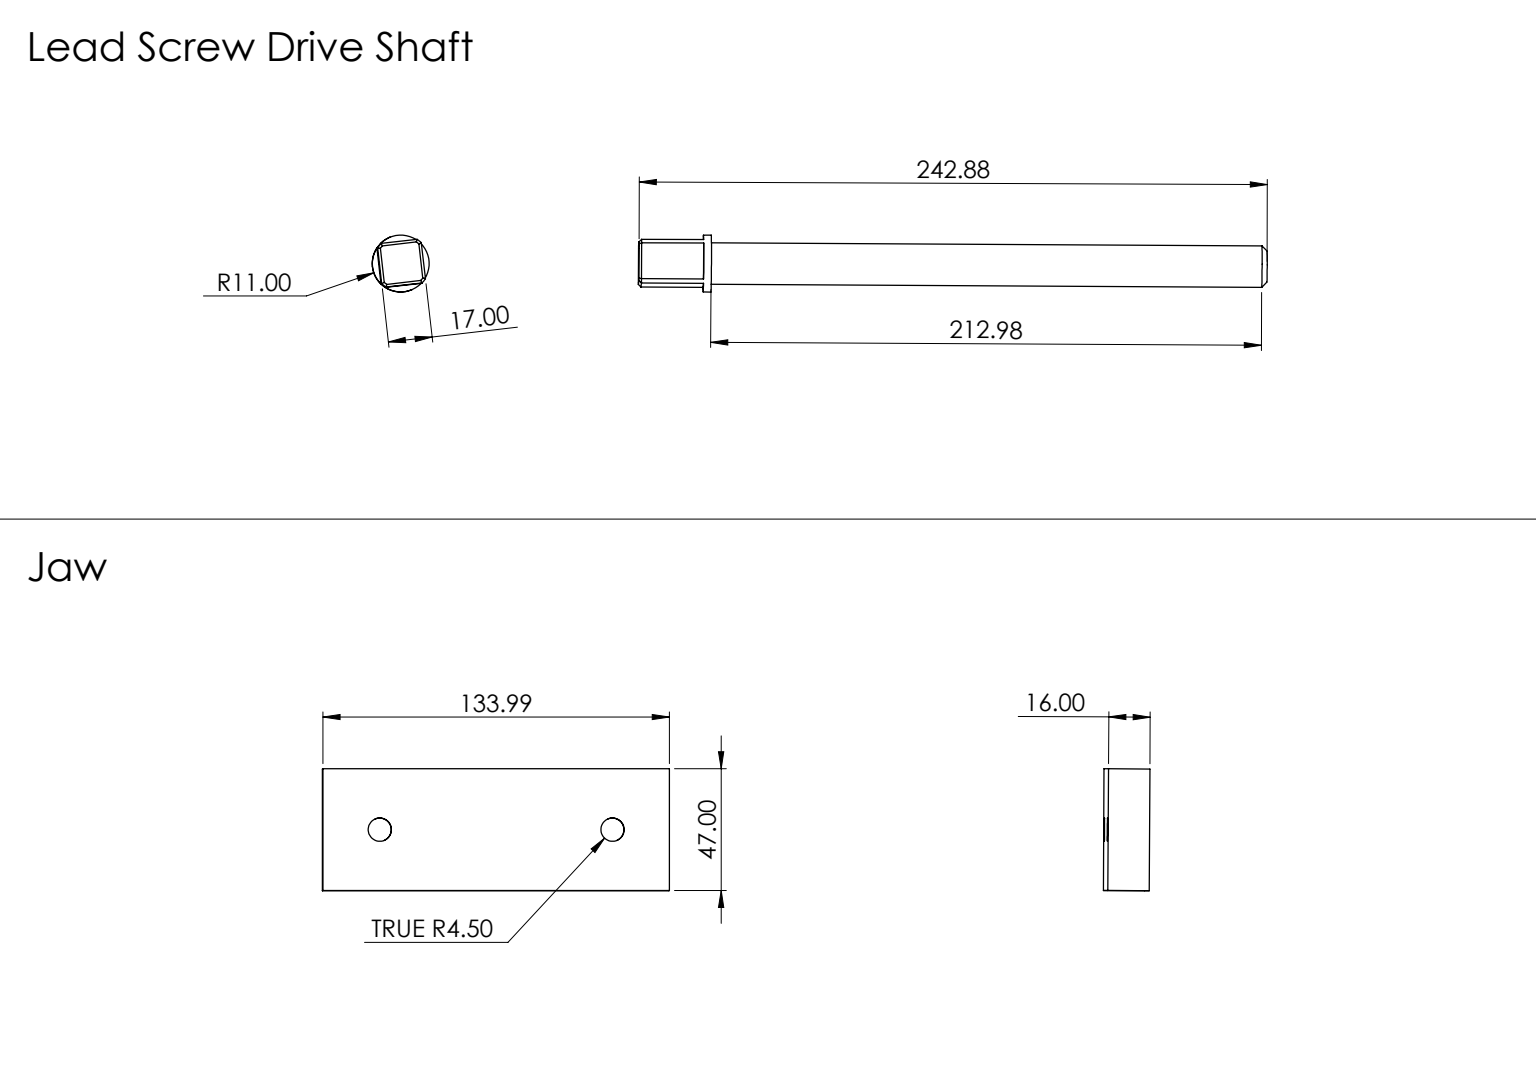
ISO-10303-21;
HEADER;
FILE_DESCRIPTION (('STEP AP214'),
    '1' );
FILE_NAME ('Lead Screw Drive Shaft.step',
    '2026-10-09T10:51:02',
    ( '' ),
    ( '' ),
    'SwSTEP 2.0',
    'SolidWorks 2026',
    '' );
FILE_SCHEMA (( 'AUTOMOTIVE_DESIGN' ));
ENDSEC;

DATA;
#4=CARTESIAN_POINT ( 'NONE',  ( 8.705884045762138257, 173.3519990577861734, 81.47578913282544022 ) ) ;
#29=EDGE_CURVE ( 'NONE', #2768, #16051, #13115, .T. ) ;
#43=AXIS2_PLACEMENT_3D ( 'NONE', #10674, #12520, #10452 ) ;
#64=DIRECTION ( 'NONE',  ( 0.9934404589540163366, 0.1135548637187051291, -0.01346653032743023830 ) ) ;
#93=EDGE_CURVE ( 'NONE', #564, #16051, #11405, .T. ) ;
#104=CIRCLE ( 'NONE', #1575, 11.00000000000000178 ) ;
#111=CARTESIAN_POINT ( 'NONE',  ( 11.83347885643962982, 174.6861507205185546, 323.4518999165990181 ) ) ;
#116=FACE_OUTER_BOUND ( 'NONE', #21594, .T. ) ;
#154=PLANE ( 'NONE',  #20182 ) ;
#206=ORIENTED_EDGE ( 'NONE', *, *, #693, .T. ) ;
#224=EDGE_LOOP ( 'NONE', ( #13231, #22623, #16630, #19910 ) ) ;
#250=DIRECTION ( 'NONE',  ( 0.01292394549866731669, 0.005513023399720593139, 0.9999012842304692006 ) ) ;
#260=DIRECTION ( 'NONE',  ( -0.9934404589540163366, -0.1135548637187053511, 0.01346653032743023309 ) ) ;
#279=FACE_BOUND ( 'NONE', #1045, .T. ) ;
#293=ORIENTED_EDGE ( 'NONE', *, *, #12181, .F. ) ;
#343=CARTESIAN_POINT ( 'NONE',  ( 11.77442667496907625, 158.9997348699313591, 299.5367818821357560 ) ) ;
#349=EDGE_CURVE ( 'NONE', #12132, #16568, #18988, .T. ) ;
#417=DIRECTION ( 'NONE',  ( 0.01292394549866731669, 0.005513023399720593139, 0.9999012842304692006 ) ) ;
#564=VERTEX_POINT ( 'NONE', #20430 ) ;
#595=ORIENTED_EDGE ( 'NONE', *, *, #9993, .F. ) ;
#640=CARTESIAN_POINT ( 'NONE',  ( 11.98277897518291013, 166.6990352492036891, 81.47011610648978319 ) ) ;
#646=CARTESIAN_POINT ( 'NONE',  ( 11.77702168924416171, 159.7711821663725971, 324.2021903088674435 ) ) ;
#675=ORIENTED_EDGE ( 'NONE', *, *, #17369, .T. ) ;
#693=EDGE_CURVE ( 'NONE', #2734, #11822, #9952, .T. ) ;
#712=EDGE_LOOP ( 'NONE', ( #4652, #19720, #8639 ) ) ;
#738=DIRECTION ( 'NONE',  ( 0.9934404589540163366, 0.1135548637187053511, -0.01346653032743023309 ) ) ;
#747=LINE ( 'NONE', #4054, #17299 ) ;
#771=PLANE ( 'NONE',  #14491 ) ;
#797=CIRCLE ( 'NONE', #1538, 11.00000000000000178 ) ;
#865=ORIENTED_EDGE ( 'NONE', *, *, #11226, .F. ) ;
#914=VECTOR ( 'NONE', #14909, 1000.000000000000114 ) ;
#942=FACE_OUTER_BOUND ( 'NONE', #11915, .T. ) ;
#1022=ORIENTED_EDGE ( 'NONE', *, *, #12685, .F. ) ;
#1045=EDGE_LOOP ( 'NONE', ( #20981, #3782 ) ) ;
#1078=ORIENTED_EDGE ( 'NONE', *, *, #12885, .T. ) ;
#1151=LINE ( 'NONE', #18927, #20877 ) ;
#1187=ORIENTED_EDGE ( 'NONE', *, *, #19016, .F. ) ;
#1189=CARTESIAN_POINT ( 'NONE',  ( -1.614838104868287605, 158.2404303229639595, 324.3837229658399792 ) ) ;
#1239=EDGE_CURVE ( 'NONE', #13001, #13489, #17742, .T. ) ;
#1325=VERTEX_POINT ( 'NONE', #16703 ) ;
#1384=PRODUCT_CONTEXT ( 'NONE', #22565, 'mechanical' ) ;
#1395=DIRECTION ( 'NONE',  ( 1.000000000000000000, 0.000000000000000000, 0.000000000000000000 ) ) ;
#1429=AXIS2_PLACEMENT_3D ( 'NONE', #11749, #10141, #6471 ) ;
#1438=DIRECTION ( 'NONE',  ( 0.01292394549866731843, 0.005513023399720594006, 0.9999012842304693116 ) ) ;
#1526=STYLED_ITEM ( 'NONE', ( #11230 ), #9502 ) ;
#1538=AXIS2_PLACEMENT_3D ( 'NONE', #8085, #15121, #22073 ) ;
#1544=CARTESIAN_POINT ( 'NONE',  ( 12.39776786404130782, 161.0697644098447370, 324.5197799491688215 ) ) ;
#1565=ADVANCED_FACE ( 'NONE', ( #19625 ), #12400, .T. ) ;
#1575=AXIS2_PLACEMENT_3D ( 'NONE', #11584, #21774, #9508 ) ;
#1609=CIRCLE ( 'NONE', #16669, 8.000000000000003553 ) ;
#1662=AXIS2_PLACEMENT_3D ( 'NONE', #19654, #14289, #2098 ) ;
#1701=CARTESIAN_POINT ( 'NONE',  ( 3.872354045398203937, 166.6517708494369856, 299.5967279023338392 ) ) ;
#1761=EDGE_CURVE ( 'NONE', #4814, #10791, #21560, .T. ) ;
#1791=ADVANCED_FACE ( 'NONE', ( #4229 ), #14606, .F. ) ;
#1795=CARTESIAN_POINT ( 'NONE',  ( -8.182603756456146016, 171.4215663745681866, 81.70472014839175756 ) ) ;
#1821=CARTESIAN_POINT ( 'NONE',  ( 3.872354045398203937, 166.6517708494369856, 299.5967279023338392 ) ) ;
#1838=CARTESIAN_POINT ( 'NONE',  ( 4.182528737366220106, 166.7840834110302808, 323.5943587238651276 ) ) ;
#1841=EDGE_CURVE ( 'NONE', #5715, #14396, #16176, .T. ) ;
#1848=CIRCLE ( 'NONE', #19071, 11.00000000000000178 ) ;
#1892=PRODUCT_DEFINITION_SHAPE ( 'NONE', 'NONE',  #18443 ) ;
#1900=AXIS2_PLACEMENT_3D ( 'NONE', #17981, #5764, #738 ) ;
#1903=CARTESIAN_POINT ( 'NONE',  ( 13.28235005706528682, 159.1720975239875884, 299.5163413053770682 ) ) ;
#1959=CIRCLE ( 'NONE', #13704, 10.00000000000005684 ) ;
#1987=CARTESIAN_POINT ( 'NONE',  ( 13.59252474903330210, 159.3044100855808836, 323.5139721269083566 ) ) ;
#1989=VERTEX_POINT ( 'NONE', #11897 ) ;
#2012=DIRECTION ( 'NONE',  ( -0.9934404589540163366, -0.1135548637187053511, 0.01346653032743023309 ) ) ;
#2016=ORIENTED_EDGE ( 'NONE', *, *, #19731, .F. ) ;
#2019=DIRECTION ( 'NONE',  ( -0.01292394549866731669, -0.005513023399720593139, -0.9999012842304692006 ) ) ;
#2022=ORIENTED_EDGE ( 'NONE', *, *, #9067, .T. ) ;
#2058=CARTESIAN_POINT ( 'NONE',  ( -4.905708827035327069, 164.7686025659857023, 81.69904712205610053 ) ) ;
#2082=ORIENTED_EDGE ( 'NONE', *, *, #20790, .F. ) ;
#2098=DIRECTION ( 'NONE',  ( -0.9934404589540177799, -0.1135548637186921672, 0.01346653032743275538 ) ) ;
#2175=VECTOR ( 'NONE', #10101, 1000.000000000000000 ) ;
#2192=CARTESIAN_POINT ( 'NONE',  ( 1.054933926688728762, 165.4499317482979279, 81.61824794009152129 ) ) ;
#2204=ORIENTED_EDGE ( 'NONE', *, *, #13338, .F. ) ;
#2244=VECTOR ( 'NONE', #7831, 1000.000000000000114 ) ;
#2266=ORIENTED_EDGE ( 'NONE', *, *, #14796, .T. ) ;
#2267=EDGE_LOOP ( 'NONE', ( #2022, #21934 ) ) ;
#2268=ORIENTED_EDGE ( 'NONE', *, *, #1239, .T. ) ;
#2283=DIRECTION ( 'NONE',  ( -0.1136178953597573732, 0.9935164314186356593, -0.004009283626633518283 ) ) ;
#2328=DIRECTION ( 'NONE',  ( 0.9934404589540162256, 0.1135548637187056842, -0.01346653032743081423 ) ) ;
#2356=EDGE_CURVE ( 'NONE', #6945, #13489, #4994, .T. ) ;
#2357=EDGE_CURVE ( 'NONE', #10791, #4814, #19010, .T. ) ;
#2442=CARTESIAN_POINT ( 'NONE',  ( 3.872354045398203937, 166.6517708494369856, 299.5967279023338392 ) ) ;
#2455=PLANE ( 'NONE',  #12630 ) ;
#2478=LINE ( 'NONE', #9473, #17026 ) ;
#2602=CARTESIAN_POINT ( 'NONE',  ( 11.61857788991896179, 160.0893180226940444, 324.5352569096220918 ) ) ;
#2712=EDGE_CURVE ( 'NONE', #4144, #14396, #9873, .T. ) ;
#2729=ORIENTED_EDGE ( 'NONE', *, *, #9691, .T. ) ;
#2734=VERTEX_POINT ( 'NONE', #15182 ) ;
#2768=VERTEX_POINT ( 'NONE', #6082 ) ;
#2788=ORIENTED_EDGE ( 'NONE', *, *, #16045, .T. ) ;
#2815=ORIENTED_EDGE ( 'NONE', *, *, #2356, .T. ) ;
#2875=DIRECTION ( 'NONE',  ( -0.9934404589540162256, -0.1135548637187059617, 0.01346653032742970747 ) ) ;
#2911=( NAMED_UNIT ( * ) SI_UNIT ( $, .STERADIAN. ) SOLID_ANGLE_UNIT ( ) );
#2931=AXIS2_PLACEMENT_3D ( 'NONE', #12386, #12833, #12495 ) ;
#2982=DIRECTION ( 'NONE',  ( -0.01292394549866731843, -0.005513023399720594006, -0.9999012842304693116 ) ) ;
#2986=CIRCLE ( 'NONE', #20594, 8.000000000000003553 ) ;
#3005=EDGE_CURVE ( 'NONE', #4814, #12132, #9983, .T. ) ;
#3008=FACE_OUTER_BOUND ( 'NONE', #10174, .T. ) ;
#3092=CIRCLE ( 'NONE', #16332, 11.00000000000000178 ) ;
#3102=CARTESIAN_POINT ( 'NONE',  ( 0.000000000000000000, 0.000000000000000000, 0.000000000000000000 ) ) ;
#3143=CARTESIAN_POINT ( 'NONE',  ( 3.872354045398203937, 166.6517708494369856, 299.5967279023338392 ) ) ;
#3166=CARTESIAN_POINT ( 'NONE',  ( -4.006862498311197562, 172.5094284590153393, 324.6687400670222701 ) ) ;
#3183=ORIENTED_EDGE ( 'NONE', *, *, #20658, .T. ) ;
#3236=AXIS2_PLACEMENT_3D ( 'NONE', #9475, #20038, #9606 ) ;
#3273=EDGE_CURVE ( 'NONE', #11778, #4144, #1151, .T. ) ;
#3297=EDGE_CURVE ( 'NONE', #16236, #13489, #8147, .T. ) ;
#3305=AXIS2_PLACEMENT_3D ( 'NONE', #18113, #22072, #20025 ) ;
#3330=ORIENTED_EDGE ( 'NONE', *, *, #21023, .F. ) ;
#3337=ADVANCED_BREP_SHAPE_REPRESENTATION ( '', ( #9502, #6292 ), #9963 ) ;
#3338=ORIENTED_EDGE ( 'NONE', *, *, #3273, .T. ) ;
#3435=CARTESIAN_POINT ( 'NONE',  ( 11.51968368760321937, 174.5313030472551645, 323.7907258472187664 ) ) ;
#3438=VERTEX_POINT ( 'NONE', #14359 ) ;
#3457=ADVANCED_FACE ( 'NONE', ( #9500 ), #5941, .T. ) ;
#3488=EDGE_LOOP ( 'NONE', ( #22441, #19131, #11485, #11826 ) ) ;
#3517=DIRECTION ( 'NONE',  ( -0.9934404589540163366, -0.1135548637187055454, 0.01346653032743023483 ) ) ;
#3554=DIRECTION ( 'NONE',  ( 0.01292394549866731669, 0.005513023399720593139, 0.9999012842304692006 ) ) ;
#3584=LINE ( 'NONE', #10593, #14733 ) ;
#3627=DIRECTION ( 'NONE',  ( -0.01292394549866731669, -0.005513023399720593139, -0.9999012842304692006 ) ) ;
#3670=EDGE_LOOP ( 'NONE', ( #16266, #5053, #5703, #9149 ) ) ;
#3704=EDGE_LOOP ( 'NONE', ( #8453, #9703 ) ) ;
#3705=UNCERTAINTY_MEASURE_WITH_UNIT (LENGTH_MEASURE( 1.000000000000000082E-05 ), #14811, 'distance_accuracy_value', 'NONE');
#3782=ORIENTED_EDGE ( 'NONE', *, *, #8180, .F. ) ;
#3784=( LENGTH_UNIT ( ) NAMED_UNIT ( * ) SI_UNIT ( .MILLI., .METRE. ) );
#3803=ORIENTED_EDGE ( 'NONE', *, *, #19177, .F. ) ;
#3808=DIRECTION ( 'NONE',  ( 0.01292394549866731669, 0.005513023399720593139, 0.9999012842304692006 ) ) ;
#3902=ORIENTED_EDGE ( 'NONE', *, *, #93, .T. ) ;
#3981=CARTESIAN_POINT ( 'NONE',  ( -4.905708827035320851, 164.7686025659857023, 81.69904712205610053 ) ) ;
#4049=CARTESIAN_POINT ( 'NONE',  ( 2.924639046024143596, 174.5833632305869401, 296.5649497806293766 ) ) ;
#4054=CARTESIAN_POINT ( 'NONE',  ( 7.025502335143726462, 174.6876751029090542, 81.49014409824067684 ) ) ;
#4111=DIRECTION ( 'NONE',  ( 0.9934404589540163366, 0.1135548637187051429, -0.01346653032743023309 ) ) ;
#4137=LINE ( 'NONE', #16125, #20508 ) ;
#4144=VERTEX_POINT ( 'NONE', #18553 ) ;
#4146=DIRECTION ( 'NONE',  ( 0.01292394549866731843, 0.005513023399720594006, 0.9999012842304693116 ) ) ;
#4202=FILL_AREA_STYLE_COLOUR ( '', #17670 ) ;
#4229=FACE_OUTER_BOUND ( 'NONE', #3704, .T. ) ;
#4261=VERTEX_POINT ( 'NONE', #5891 ) ;
#4300=ADVANCED_FACE ( 'NONE', ( #13709 ), #8394, .T. ) ;
#4302=FACE_OUTER_BOUND ( 'NONE', #712, .T. ) ;
#4313=ORIENTED_EDGE ( 'NONE', *, *, #19177, .T. ) ;
#4323=DIRECTION ( 'NONE',  ( -0.9934404589540162256, -0.1135548637187059617, 0.01346653032743144220 ) ) ;
#4332=DIRECTION ( 'NONE',  ( 0.9934404589540163366, 0.1135548637187057675, -0.01346653032742924257 ) ) ;
#4339=ADVANCED_FACE ( 'NONE', ( #3008 ), #16932, .T. ) ;
#4392=EDGE_LOOP ( 'NONE', ( #6382, #2016, #18881, #20191 ) ) ;
#4490=ADVANCED_FACE ( 'NONE', ( #19448 ), #7662, .T. ) ;
#4494=CARTESIAN_POINT ( 'NONE',  ( -1.702894481557716944, 157.8934747572109814, 324.0533643900782295 ) ) ;
#4652=ORIENTED_EDGE ( 'NONE', *, *, #14489, .T. ) ;
#4698=AXIS2_PLACEMENT_3D ( 'NONE', #11868, #13482, #22500 ) ;
#4730=SURFACE_STYLE_FILL_AREA ( #15342 ) ;
#4814=VERTEX_POINT ( 'NONE', #14928 ) ;
#4831=DIRECTION ( 'NONE',  ( 0.01292394549866731843, 0.005513023399720594006, 0.9999012842304693116 ) ) ;
#4870=CARTESIAN_POINT ( 'NONE',  ( -4.113941462729931331, 165.7267928694881789, 296.7047562922618908 ) ) ;
#4977=ORIENTED_EDGE ( 'NONE', *, *, #15833, .F. ) ;
#4980=CARTESIAN_POINT ( 'NONE',  ( 4.182528737366220106, 166.7840834110302808, 323.5943587238651276 ) ) ;
#4983=APPLICATION_CONTEXT ( 'automotive_design' ) ;
#4994=B_SPLINE_CURVE_WITH_KNOTS ( 'NONE', 3,
 ( #15322, #1189, #4494, #16811 ),
 .UNSPECIFIED., .F., .F.,
 ( 4, 4 ),
 ( 0.000000000000000000, 0.001461243987307916069 ),
 .UNSPECIFIED. ) ;
#5053=ORIENTED_EDGE ( 'NONE', *, *, #15833, .T. ) ;
#5104=DIRECTION ( 'NONE',  ( 0.01292394549866731669, 0.005513023399720593139, 0.9999012842304692006 ) ) ;
#5206=PLANE ( 'NONE',  #19572 ) ;
#5260=CONICAL_SURFACE ( 'NONE', #18147, 11.00000000000000178, 0.7853981633974346233 ) ;
#5285=ADVANCED_FACE ( 'NONE', ( #19749 ), #11046, .T. ) ;
#5290=DIRECTION ( 'NONE',  ( -0.9934404589540172248, -0.1135548637186977322, 0.01346653032743275885 ) ) ;
#5330=EDGE_CURVE ( 'NONE', #11842, #1325, #4137, .T. ) ;
#5375=CARTESIAN_POINT ( 'NONE',  ( 9.914309459522627321, 174.9920644939733734, 324.4751176552225616 ) ) ;
#5376=CARTESIAN_POINT ( 'NONE',  ( 1.054933926688728762, 165.4499317482979279, 81.61824794009152129 ) ) ;
#5382=DIRECTION ( 'NONE',  ( -0.9934404589540162256, -0.1135548637187056842, 0.01346653032743081423 ) ) ;
#5503=CARTESIAN_POINT ( 'NONE',  ( 4.182528737366220106, 166.7840834110302808, 323.5943587238651276 ) ) ;
#5518=DIRECTION ( 'NONE',  ( -0.9934404589540162256, -0.1135548637187056842, 0.01346653032743081423 ) ) ;
#5554=FACE_OUTER_BOUND ( 'NONE', #18914, .T. ) ;
#5646=CARTESIAN_POINT ( 'NONE',  ( 3.872354045398203937, 166.6517708494369856, 299.5967279023338392 ) ) ;
#5693=LINE ( 'NONE', #19364, #7860 ) ;
#5703=ORIENTED_EDGE ( 'NONE', *, *, #349, .T. ) ;
#5715=VERTEX_POINT ( 'NONE', #19136 ) ;
#5764=DIRECTION ( 'NONE',  ( -0.08947859377482220156, 0.6986239096456045017, -0.7098719702365846596 ) ) ;
#5846=EDGE_CURVE ( 'NONE', #16236, #18202, #19440, .T. ) ;
#5890=PLANE ( 'NONE',  #1900 ) ;
#5891=CARTESIAN_POINT ( 'NONE',  ( -7.055491003095976765, 165.4026673485312244, 299.7448597359355631 ) ) ;
#5941=PLANE ( 'NONE',  #10624 ) ;
#6029=VECTOR ( 'NONE', #19401, 1000.000000000000227 ) ;
#6041=CARTESIAN_POINT ( 'NONE',  ( 12.08460136693709153, 159.1320474315246543, 323.5344127036669875 ) ) ;
#6082=CARTESIAN_POINT ( 'NONE',  ( 12.39776786404130782, 161.0697644098447370, 324.5197799491688215 ) ) ;
#6138=CARTESIAN_POINT ( 'NONE',  ( -2.098214363056787768, 157.4140274948258593, 299.7248317441846552 ) ) ;
#6145=CARTESIAN_POINT ( 'NONE',  ( -3.719543892204659752, 174.4361193905359642, 323.6543047440632108 ) ) ;
#6148=EDGE_CURVE ( 'NONE', #1989, #13001, #1848, .T. ) ;
#6193=DIRECTION ( 'NONE',  ( -0.01292394549866731843, -0.005513023399720594006, -0.9999012842304693116 ) ) ;
#6221=EDGE_LOOP ( 'NONE', ( #14252, #14224, #13123, #7707 ) ) ;
#6277=CARTESIAN_POINT ( 'NONE',  ( -4.505147608247620283, 176.8666157021447134, 324.6511568656583222 ) ) ;
#6292=AXIS2_PLACEMENT_3D ( 'NONE', #3102, #12069, #1395 ) ;
#6296=ORIENTED_EDGE ( 'NONE', *, *, #11840, .F. ) ;
#6315=B_SPLINE_CURVE_WITH_KNOTS ( 'NONE', 3,
 ( #22476, #17228, #15638, #8598 ),
 .UNSPECIFIED., .F., .F.,
 ( 4, 4 ),
 ( 0.000000000000000000, 0.001461243987307901107 ),
 .UNSPECIFIED. ) ;
#6324=SHAPE_DEFINITION_REPRESENTATION ( #1892, #9590 ) ;
#6349=ORIENTED_EDGE ( 'NONE', *, *, #13250, .F. ) ;
#6356=FACE_OUTER_BOUND ( 'NONE', #4392, .T. ) ;
#6369=B_SPLINE_CURVE_WITH_KNOTS ( 'NONE', 3,
 ( #16301, #646, #7634, #6041 ),
 .UNSPECIFIED., .F., .F.,
 ( 4, 4 ),
 ( 0.000000000000000000, 0.001461243987308225717 ),
 .UNSPECIFIED. ) ;
#6382=ORIENTED_EDGE ( 'NONE', *, *, #20850, .T. ) ;
#6411=VECTOR ( 'NONE', #6634, 1000.000000000000227 ) ;
#6419=AXIS2_PLACEMENT_3D ( 'NONE', #15516, #11946, #6645 ) ;
#6471=DIRECTION ( 'NONE',  ( -0.9934404589540162256, -0.1135548637187056842, 0.01346653032743081423 ) ) ;
#6484=( NAMED_UNIT ( * ) PLANE_ANGLE_UNIT ( ) SI_UNIT ( $, .RADIAN. ) );
#6526=EDGE_CURVE ( 'NONE', #13001, #18202, #3584, .T. ) ;
#6538=ADVANCED_FACE ( 'NONE', ( #16026 ), #154, .T. ) ;
#6602=DIRECTION ( 'NONE',  ( -0.01292394549866731843, -0.005513023399720594006, -0.9999012842304693116 ) ) ;
#6634=DIRECTION ( 'NONE',  ( 0.1136178953597573593, -0.9935164314186355483, 0.004009283626633517415 ) ) ;
#6637=LINE ( 'NONE', #16926, #22034 ) ;
#6642=CARTESIAN_POINT ( 'NONE',  ( -4.915634481766264052, 156.2121883936867732, 81.74635178194236573 ) ) ;
#6645=DIRECTION ( 'NONE',  ( -0.9934404589540162256, -0.1135548637187060589, 0.01346653032743275885 ) ) ;
#6738=EDGE_CURVE ( 'NONE', #10848, #5715, #6637, .T. ) ;
#6739=EDGE_LOOP ( 'NONE', ( #206, #15187, #6296 ) ) ;
#6774=CIRCLE ( 'NONE', #22519, 11.00000000000000178 ) ;
#6823=DIRECTION ( 'NONE',  ( 0.01292394549866731843, 0.005513023399720594006, 0.9999012842304693116 ) ) ;
#6831=B_SPLINE_CURVE_WITH_KNOTS ( 'NONE', 3,
 ( #13717, #8074, #11878, #13599 ),
 .UNSPECIFIED., .F., .F.,
 ( 4, 4 ),
 ( 0.000000000000000000, 0.001461243987308210755 ),
 .UNSPECIFIED. ) ;
#6833=CARTESIAN_POINT ( 'NONE',  ( -9.872911121805453050, 164.2008282473921668, 81.76637977369325938 ) ) ;
#6945=VERTEX_POINT ( 'NONE', #8920 ) ;
#6969=DIRECTION ( 'NONE',  ( -0.9934404589540162256, -0.1135548637187055315, 0.01346653032743023309 ) ) ;
#7006=DIRECTION ( 'NONE',  ( 0.01292394549866731669, 0.005513023399720593139, 0.9999012842304692006 ) ) ;
#7024=CARTESIAN_POINT ( 'NONE',  ( -3.778596073675196454, 158.7497035399487402, 299.7391867095999487 ) ) ;
#7107=FACE_OUTER_BOUND ( 'NONE', #15836, .T. ) ;
#7109=EDGE_CURVE ( 'NONE', #20855, #22352, #2986, .T. ) ;
#7122=ADVANCED_FACE ( 'NONE', ( #14538 ), #5890, .F. ) ;
#7140=( GEOMETRIC_REPRESENTATION_CONTEXT ( 3 ) GLOBAL_UNCERTAINTY_ASSIGNED_CONTEXT ( ( #3705 ) ) GLOBAL_UNIT_ASSIGNED_CONTEXT ( ( #14811, #6484, #2911 ) ) REPRESENTATION_CONTEXT ( 'NONE', 'WORKASPACE' ) );
#7152=CIRCLE ( 'NONE', #6419, 10.00000000000005684 ) ;
#7153=DIRECTION ( 'NONE',  ( 0.9934404589540163366, 0.1135548637187051429, -0.01346653032743023309 ) ) ;
#7272=DIRECTION ( 'NONE',  ( -0.01292394549866731843, -0.005513023399720594006, -0.9999012842304693116 ) ) ;
#7359=DIRECTION ( 'NONE',  ( -0.9934404589540162256, -0.1135548637187055315, 0.01346653032743023309 ) ) ;
#7385=DIRECTION ( 'NONE',  ( -0.01292394549866731843, -0.005513023399720594006, -0.9999012842304693116 ) ) ;
#7413=AXIS2_PLACEMENT_3D ( 'NONE', #1701, #18813, #11694 ) ;
#7439=ORIENTED_EDGE ( 'NONE', *, *, #17369, .F. ) ;
#7486=EDGE_LOOP ( 'NONE', ( #4977, #14173, #10435, #14164 ) ) ;
#7576=ADVANCED_FACE ( 'NONE', ( #8966 ), #12188, .T. ) ;
#7608=ORIENTED_EDGE ( 'NONE', *, *, #8776, .F. ) ;
#7634=CARTESIAN_POINT ( 'NONE',  ( 11.93221611429111384, 159.4520312983160295, 323.8685343595495851 ) ) ;
#7662=CONICAL_SURFACE ( 'NONE', #14669, 11.00000000000000178, 0.7853981633974346233 ) ;
#7677=CARTESIAN_POINT ( 'NONE',  ( 1.054933926688728762, 165.4499317482979279, 81.61824794009152129 ) ) ;
#7707=ORIENTED_EDGE ( 'NONE', *, *, #3005, .F. ) ;
#7745=AXIS2_PLACEMENT_3D ( 'NONE', #20956, #64, #2019 ) ;
#7773=SURFACE_SIDE_STYLE ('',( #4730 ) ) ;
#7798=ORIENTED_EDGE ( 'NONE', *, *, #9691, .F. ) ;
#7801=CARTESIAN_POINT ( 'NONE',  ( 1.054933926688728762, 165.4499317482979279, 81.61824794009152129 ) ) ;
#7831=DIRECTION ( 'NONE',  ( -0.01292394549866731669, -0.005513023399720593139, -0.9999012842304692006 ) ) ;
#7839=AXIS2_PLACEMENT_3D ( 'NONE', #4980, #6602, #18997 ) ;
#7860=VECTOR ( 'NONE', #3627, 1000.000000000000114 ) ;
#7871=LINE ( 'NONE', #640, #914 ) ;
#7921=CONICAL_SURFACE ( 'NONE', #14185, 11.00000000000000178, 0.7853981633974346233 ) ;
#7924=ADVANCED_FACE ( 'NONE', ( #10112 ), #15303, .F. ) ;
#7979=ORIENTED_EDGE ( 'NONE', *, *, #5846, .T. ) ;
#7999=VECTOR ( 'NONE', #417, 1000.000000000000114 ) ;
#8074=CARTESIAN_POINT ( 'NONE',  ( -2.824407579846267335, 159.2018743582275988, 324.3940559323744424 ) ) ;
#8085=CARTESIAN_POINT ( 'NONE',  ( 3.872354045398203937, 166.6517708494369856, 299.5967279023338392 ) ) ;
#8110=DIRECTION ( 'NONE',  ( 0.9934404589540163366, 0.1135548637187051429, -0.01346653032743023309 ) ) ;
#8122=ADVANCED_FACE ( 'NONE', ( #7107 ), #16212, .T. ) ;
#8147=LINE ( 'NONE', #6642, #10986 ) ;
#8158=DIRECTION ( 'NONE',  ( -0.01292394549866731669, -0.005513023399720593139, -0.9999012842304692006 ) ) ;
#8180=EDGE_CURVE ( 'NONE', #22352, #20855, #21001, .T. ) ;
#8308=CARTESIAN_POINT ( 'NONE',  ( 13.42006642051110177, 160.8124487847600221, 323.5078865155649055 ) ) ;
#8394=CYLINDRICAL_SURFACE ( 'NONE', #4698, 8.000000000000003553 ) ;
#8414=ORIENTED_EDGE ( 'NONE', *, *, #29, .F. ) ;
#8440=ORIENTED_EDGE ( 'NONE', *, *, #20658, .F. ) ;
#8453=ORIENTED_EDGE ( 'NONE', *, *, #1761, .T. ) ;
#8473=CARTESIAN_POINT ( 'NONE',  ( 13.28235005706528682, 159.1720975239875884, 299.5163413053770682 ) ) ;
#8514=VECTOR ( 'NONE', #18949, 1000.000000000000227 ) ;
#8564=CARTESIAN_POINT ( 'NONE',  ( 12.08460136693709153, 159.1320474315246543, 323.5344127036669875 ) ) ;
#8597=ORIENTED_EDGE ( 'NONE', *, *, #20137, .F. ) ;
#8598=CARTESIAN_POINT ( 'NONE',  ( -5.055008945778654450, 172.7557180373005679, 323.6808309321652928 ) ) ;
#8638=ORIENTED_EDGE ( 'NONE', *, *, #14489, .F. ) ;
#8639=ORIENTED_EDGE ( 'NONE', *, *, #12685, .T. ) ;
#8650=PRODUCT ( 'Lead Screw Drive Shaft', 'Lead Screw Drive Shaft', '', ( #1384 ) ) ;
#8718=ORIENTED_EDGE ( 'NONE', *, *, #1841, .T. ) ;
#8776=EDGE_CURVE ( 'NONE', #4261, #12198, #19003, .T. ) ;
#8821=CARTESIAN_POINT ( 'NONE',  ( 4.182528737366220106, 166.7840834110302808, 323.5943587238651276 ) ) ;
#8827=( NAMED_UNIT ( * ) PLANE_ANGLE_UNIT ( ) SI_UNIT ( $, .RADIAN. ) );
#8920=CARTESIAN_POINT ( 'NONE',  ( -1.523404093792848135, 158.5871283748866745, 324.7134023609685869 ) ) ;
#8945=( NAMED_UNIT ( * ) SI_UNIT ( $, .STERADIAN. ) SOLID_ANGLE_UNIT ( ) );
#8966=FACE_OUTER_BOUND ( 'NONE', #18599, .T. ) ;
#8995=DIRECTION ( 'NONE',  ( -0.9934404589540162256, -0.1135548637187059617, 0.01346653032743144220 ) ) ;
#9067=EDGE_CURVE ( 'NONE', #12198, #3438, #11407, .T. ) ;
#9072=ORIENTED_EDGE ( 'NONE', *, *, #22132, .F. ) ;
#9108=DIRECTION ( 'NONE',  ( -0.1136178953597575675, 0.9935164314186356593, -0.004009283626633515681 ) ) ;
#9136=CARTESIAN_POINT ( 'NONE',  ( 10.15309714582121714, 176.0218267656414355, 323.4662548820142547 ) ) ;
#9149=ORIENTED_EDGE ( 'NONE', *, *, #10055, .F. ) ;
#9158=LINE ( 'NONE', #3981, #18804 ) ;
#9273=DIRECTION ( 'NONE',  ( -0.9934404589540163366, -0.1135548637187055454, 0.01346653032743023483 ) ) ;
#9289=ORIENTED_EDGE ( 'NONE', *, *, #6738, .F. ) ;
#9300=EDGE_LOOP ( 'NONE', ( #8718, #14452, #21930, #14298 ) ) ;
#9401=DIRECTION ( 'NONE',  ( -0.01292394549866731843, -0.005513023399720594006, -0.9999012842304693116 ) ) ;
#9463=VERTEX_POINT ( 'NONE', #17161 ) ;
#9473=CARTESIAN_POINT ( 'NONE',  ( 10.15309714582121714, 176.0218267656414355, 323.4662548820142547 ) ) ;
#9475=CARTESIAN_POINT ( 'NONE',  ( 1.080781817686064405, 165.4609577950973573, 83.61805050855254251 ) ) ;
#9500=FACE_OUTER_BOUND ( 'NONE', #9300, .T. ) ;
#9502=MANIFOLD_SOLID_BREP ( 'Stock-MAS-425-1', #21953 ) ;
#9508=DIRECTION ( 'NONE',  ( 0.9934404589540162256, 0.1135548637187056842, -0.01346653032743081423 ) ) ;
#9528=ORIENTED_EDGE ( 'NONE', *, *, #6148, .T. ) ;
#9529=UNCERTAINTY_MEASURE_WITH_UNIT (LENGTH_MEASURE( 1.000000000000000082E-05 ), #3784, 'distance_accuracy_value', 'NONE');
#9590=SHAPE_REPRESENTATION ( 'Lead Screw Drive Shaft', ( #6292 ), #9963 ) ;
#9606=DIRECTION ( 'NONE',  ( 0.9934404589540162256, 0.1135548637187059617, -0.01346653032742970747 ) ) ;
#9658=B_SPLINE_CURVE_WITH_KNOTS ( 'NONE', 3,
 ( #19505, #21470, #15628, #21518 ),
 .UNSPECIFIED., .F., .F.,
 ( 4, 4 ),
 ( 0.000000000000000000, 0.001461243987307977218 ),
 .UNSPECIFIED. ) ;
#9670=EDGE_CURVE ( 'NONE', #4261, #17346, #6774, .T. ) ;
#9691=EDGE_CURVE ( 'NONE', #1325, #12915, #11564, .T. ) ;
#9703=ORIENTED_EDGE ( 'NONE', *, *, #2357, .T. ) ;
#9742=ORIENTED_EDGE ( 'NONE', *, *, #20790, .T. ) ;
#9766=CARTESIAN_POINT ( 'NONE',  ( 4.182528737366220106, 166.7840834110302808, 323.5943587238651276 ) ) ;
#9784=FACE_OUTER_BOUND ( 'NONE', #3670, .T. ) ;
#9795=DIRECTION ( 'NONE',  ( -0.01292394549866731843, -0.005513023399720594006, -0.9999012842304693116 ) ) ;
#9873=CIRCLE ( 'NONE', #12078, 11.00000000000000178 ) ;
#9952=CIRCLE ( 'NONE', #43, 11.00000000000000178 ) ;
#9963=( GEOMETRIC_REPRESENTATION_CONTEXT ( 3 ) GLOBAL_UNCERTAINTY_ASSIGNED_CONTEXT ( ( #9529 ) ) GLOBAL_UNIT_ASSIGNED_CONTEXT ( ( #3784, #8827, #8945 ) ) REPRESENTATION_CONTEXT ( 'NONE', 'WORKASPACE' ) );
#9983=LINE ( 'NONE', #11830, #2175 ) ;
#9993=EDGE_CURVE ( 'NONE', #15528, #564, #15760, .T. ) ;
#10055=EDGE_CURVE ( 'NONE', #20855, #16568, #15999, .T. ) ;
#10101=DIRECTION ( 'NONE',  ( 0.7116070947332493457, 0.08419371040299269970, 0.6975147036829268954 ) ) ;
#10112=FACE_OUTER_BOUND ( 'NONE', #19507, .T. ) ;
#10134=DIRECTION ( 'NONE',  ( 0.9934404589540163366, 0.1135548637187057675, -0.01346653032742924257 ) ) ;
#10141=DIRECTION ( 'NONE',  ( -0.01292394549866731843, -0.005513023399720594006, -0.9999012842304693116 ) ) ;
#10174=EDGE_LOOP ( 'NONE', ( #14222, #21310, #8440, #9528, #16260, #19726, #11548, #1078, #11985, #15523, #20352, #2204 ) ) ;
#10192=ORIENTED_EDGE ( 'NONE', *, *, #14369, .T. ) ;
#10208=DIRECTION ( 'NONE',  ( 0.01292394549866731669, 0.005513023399720593139, 0.9999012842304692006 ) ) ;
#10219=DIRECTION ( 'NONE',  ( 0.9934404589540163366, 0.1135548637187051291, -0.01346653032743023830 ) ) ;
#10392=EDGE_LOOP ( 'NONE', ( #15066, #3338, #17673, #1022 ) ) ;
#10435=ORIENTED_EDGE ( 'NONE', *, *, #10055, .T. ) ;
#10452=DIRECTION ( 'NONE',  ( 0.9934404589540162256, 0.1135548637187056842, -0.01346653032743081423 ) ) ;
#10465=ADVANCED_FACE ( 'NONE', ( #942 ), #16385, .T. ) ;
#10538=CARTESIAN_POINT ( 'NONE',  ( 9.028305489318197985, 166.3693967048470199, 83.51031826593310825 ) ) ;
#10593=CARTESIAN_POINT ( 'NONE',  ( 8.957006556259601737, 157.7978957687922446, 81.55830191989343803 ) ) ;
#10612=ADVANCED_FACE ( 'NONE', ( #116 ), #7921, .T. ) ;
#10615=EDGE_CURVE ( 'NONE', #12915, #4144, #6315, .T. ) ;
#10624=AXIS2_PLACEMENT_3D ( 'NONE', #19943, #16425, #9273 ) ;
#10666=DIRECTION ( 'NONE',  ( -0.6933298757296632031, -0.07639711794142747814, 0.7165592535100873128 ) ) ;
#10674=CARTESIAN_POINT ( 'NONE',  ( 3.872354045398203937, 166.6517708494369856, 299.5967279023338392 ) ) ;
#10791=VERTEX_POINT ( 'NONE', #2058 ) ;
#10824=VERTEX_POINT ( 'NONE', #2602 ) ;
#10848=VERTEX_POINT ( 'NONE', #20829 ) ;
#10860=DIRECTION ( 'NONE',  ( -0.9934404589540162256, -0.1135548637187056842, 0.01346653032743081423 ) ) ;
#10866=ORIENTED_EDGE ( 'NONE', *, *, #10615, .T. ) ;
#10949=EDGE_CURVE ( 'NONE', #20688, #564, #22104, .T. ) ;
#10954=CARTESIAN_POINT ( 'NONE',  ( -1.788039671088772931, 157.5463400564191545, 323.7224625657159436 ) ) ;
#10973=ADVANCED_FACE ( 'NONE', ( #5554 ), #14438, .F. ) ;
#10986=VECTOR ( 'NONE', #10208, 1000.000000000000114 ) ;
#11006=CARTESIAN_POINT ( 'NONE',  ( 13.59252474903330210, 159.3044100855808836, 323.5139721269083566 ) ) ;
#11046=CYLINDRICAL_SURFACE ( 'NONE', #11728, 11.00000000000000178 ) ;
#11122=AXIS2_PLACEMENT_3D ( 'NONE', #16766, #14824, #4323 ) ;
#11130=FACE_OUTER_BOUND ( 'NONE', #6739, .T. ) ;
#11146=AXIS2_PLACEMENT_3D ( 'NONE', #19450, #13951, #15689 ) ;
#11226=EDGE_CURVE ( 'NONE', #19373, #11778, #6831, .T. ) ;
#11230=PRESENTATION_STYLE_ASSIGNMENT (( #18760 ) ) ;
#11369=DIRECTION ( 'NONE',  ( -0.9934404589540162256, -0.1135548637187056842, 0.01346653032743081423 ) ) ;
#11397=ORIENTED_EDGE ( 'NONE', *, *, #19731, .T. ) ;
#11403=AXIS2_PLACEMENT_3D ( 'NONE', #8473, #10219, #8158 ) ;
#11405=B_SPLINE_CURVE_WITH_KNOTS ( 'NONE', 3,
 ( #111, #3435, #19045, #17348 ),
 .UNSPECIFIED., .F., .F.,
 ( 4, 4 ),
 ( 0.000000000000000000, 0.001461243987307979820 ),
 .UNSPECIFIED. ) ;
#11407=CIRCLE ( 'NONE', #3305, 11.00000000000000178 ) ;
#11432=LINE ( 'NONE', #16736, #17044 ) ;
#11485=ORIENTED_EDGE ( 'NONE', *, *, #20850, .F. ) ;
#11504=CIRCLE ( 'NONE', #16657, 11.00000000000000178 ) ;
#11525=CARTESIAN_POINT ( 'NONE',  ( 1.054933926688728762, 165.4499317482979279, 81.61824794009152129 ) ) ;
#11548=ORIENTED_EDGE ( 'NONE', *, *, #3297, .T. ) ;
#11564=CIRCLE ( 'NONE', #1662, 10.00000000000005862 ) ;
#11578=VECTOR ( 'NONE', #21350, 1000.000000000000114 ) ;
#11584=CARTESIAN_POINT ( 'NONE',  ( 3.872354045398203937, 166.6517708494369856, 299.5967279023338392 ) ) ;
#11668=DIRECTION ( 'NONE',  ( -0.9934404589540162256, -0.1135548637187060589, 0.01346653032743275885 ) ) ;
#11694=DIRECTION ( 'NONE',  ( 0.9934404589540163366, 0.1135548637187051429, -0.01346653032743023309 ) ) ;
#11728=AXIS2_PLACEMENT_3D ( 'NONE', #2192, #16363, #5518 ) ;
#11749=CARTESIAN_POINT ( 'NONE',  ( 1.054933926688728762, 165.4499317482979279, 81.61824794009152129 ) ) ;
#11778=VERTEX_POINT ( 'NONE', #17477 ) ;
#11822=VERTEX_POINT ( 'NONE', #12311 ) ;
#11826=ORIENTED_EDGE ( 'NONE', *, *, #13184, .F. ) ;
#11830=CARTESIAN_POINT ( 'NONE',  ( 7.015576680412777932, 166.1312609306101535, 81.53744875812694204 ) ) ;
#11831=CARTESIAN_POINT ( 'NONE',  ( 9.002457598320861010, 166.3583706580475621, 81.51051569747208703 ) ) ;
#11840=EDGE_CURVE ( 'NONE', #2734, #15528, #15876, .T. ) ;
#11842=VERTEX_POINT ( 'NONE', #5375 ) ;
#11868=CARTESIAN_POINT ( 'NONE',  ( 1.054933926688728762, 165.4499317482979279, 81.61824794009152129 ) ) ;
#11878=CARTESIAN_POINT ( 'NONE',  ( -3.145996032882572457, 159.0405451880567682, 324.0656923467140018 ) ) ;
#11897=CARTESIAN_POINT ( 'NONE',  ( 13.42006642051110177, 160.8124487847600221, 323.5078865155649055 ) ) ;
#11915=EDGE_LOOP ( 'NONE', ( #14327, #7439, #17974, #13355 ) ) ;
#11946=DIRECTION ( 'NONE',  ( 0.01292394549866731843, 0.005513023399720594006, 0.9999012842304693116 ) ) ;
#11985=ORIENTED_EDGE ( 'NONE', *, *, #22525, .T. ) ;
#12011=CARTESIAN_POINT ( 'NONE',  ( 9.997142846107600178, 175.3350937402613852, 324.1393829572561458 ) ) ;
#12069=DIRECTION ( 'NONE',  ( 0.000000000000000000, 0.000000000000000000, 1.000000000000000000 ) ) ;
#12078=AXIS2_PLACEMENT_3D ( 'NONE', #9766, #6193, #11369 ) ;
#12132=VERTEX_POINT ( 'NONE', #10538 ) ;
#12153=CARTESIAN_POINT ( 'NONE',  ( -7.094262839591980452, 165.3861282783320803, 296.7451558832441378 ) ) ;
#12161=DIRECTION ( 'NONE',  ( -0.01292394549866731669, -0.005513023399720593139, -0.9999012842304692006 ) ) ;
#12181=EDGE_CURVE ( 'NONE', #564, #1989, #22337, .T. ) ;
#12188=CONICAL_SURFACE ( 'NONE', #17707, 5.999999999999951150, 0.7853981633974415066 ) ;
#12198=VERTEX_POINT ( 'NONE', #12153 ) ;
#12246=CARTESIAN_POINT ( 'NONE',  ( 10.07658213627836119, 175.6783734781009798, 323.8030538038543682 ) ) ;
#12266=CARTESIAN_POINT ( 'NONE',  ( -2.503839020269049254, 159.3664414540641587, 324.7217779040802270 ) ) ;
#12311=CARTESIAN_POINT ( 'NONE',  ( 14.80019909389238464, 167.9008743503427468, 299.4485960687320585 ) ) ;
#12340=DIRECTION ( 'NONE',  ( 0.01292394549866731149, 0.005513023399720593139, 0.9999012842304692006 ) ) ;
#12386=CARTESIAN_POINT ( 'NONE',  ( 3.872354045398203937, 166.6517708494369856, 299.5967279023338392 ) ) ;
#12400=CONICAL_SURFACE ( 'NONE', #12772, 5.999999999999951150, 0.7853981633974415066 ) ;
#12417=AXIS2_PLACEMENT_3D ( 'NONE', #7677, #21558, #4111 ) ;
#12429=DIRECTION ( 'NONE',  ( 0.9934404589540163366, 0.1135548637187057813, -0.01346653032742924430 ) ) ;
#12495=DIRECTION ( 'NONE',  ( 0.9934404589540162256, 0.1135548637187056842, -0.01346653032743081423 ) ) ;
#12512=VECTOR ( 'NONE', #13854, 1000.000000000000114 ) ;
#12520=DIRECTION ( 'NONE',  ( 0.01292394549866731843, 0.005513023399720594006, 0.9999012842304693116 ) ) ;
#12579=CARTESIAN_POINT ( 'NONE',  ( 4.182528737366220106, 166.7840834110302808, 323.5943587238651276 ) ) ;
#12630=AXIS2_PLACEMENT_3D ( 'NONE', #16488, #14776, #21728 ) ;
#12659=ORIENTED_EDGE ( 'NONE', *, *, #1239, .F. ) ;
#12685=EDGE_CURVE ( 'NONE', #17346, #9463, #20342, .T. ) ;
#12701=AXIS2_PLACEMENT_3D ( 'NONE', #13457, #2982, #20088 ) ;
#12772=AXIS2_PLACEMENT_3D ( 'NONE', #5376, #3554, #17360 ) ;
#12815=ORIENTED_EDGE ( 'NONE', *, *, #5330, .T. ) ;
#12833=DIRECTION ( 'NONE',  ( 0.01292394549866731843, 0.005513023399720594006, 0.9999012842304693116 ) ) ;
#12885=EDGE_CURVE ( 'NONE', #13489, #11778, #11504, .T. ) ;
#12915=VERTEX_POINT ( 'NONE', #3166 ) ;
#12948=DIRECTION ( 'NONE',  ( 0.9934404589540163366, 0.1135548637187053511, -0.01346653032743023309 ) ) ;
#12960=AXIS2_PLACEMENT_3D ( 'NONE', #1821, #18034, #16210 ) ;
#12961=DIRECTION ( 'NONE',  ( 0.1136178953597573593, -0.9935164314186355483, 0.004009283626633517415 ) ) ;
#12985=VECTOR ( 'NONE', #20085, 1000.000000000000227 ) ;
#13001=VERTEX_POINT ( 'NONE', #8564 ) ;
#13015=B_SPLINE_CURVE_WITH_KNOTS ( 'NONE', 3,
 ( #22637, #12246, #12011, #20614 ),
 .UNSPECIFIED., .F., .F.,
 ( 4, 4 ),
 ( 0.000000000000000000, 0.001461243987308227452 ),
 .UNSPECIFIED. ) ;
#13060=EDGE_CURVE ( 'NONE', #9463, #4144, #14219, .T. ) ;
#13115=LINE ( 'NONE', #18504, #12985 ) ;
#13123=ORIENTED_EDGE ( 'NONE', *, *, #349, .F. ) ;
#13157=FACE_OUTER_BOUND ( 'NONE', #3488, .T. ) ;
#13184=EDGE_CURVE ( 'NONE', #14396, #20688, #2478, .T. ) ;
#13225=ORIENTED_EDGE ( 'NONE', *, *, #1761, .F. ) ;
#13231=ORIENTED_EDGE ( 'NONE', *, *, #11226, .T. ) ;
#13250=EDGE_CURVE ( 'NONE', #10824, #13001, #6369, .T. ) ;
#13338=EDGE_CURVE ( 'NONE', #3438, #12198, #13726, .T. ) ;
#13355=ORIENTED_EDGE ( 'NONE', *, *, #6148, .F. ) ;
#13359=CYLINDRICAL_SURFACE ( 'NONE', #19110, 8.000000000000003553 ) ;
#13385=ORIENTED_EDGE ( 'NONE', *, *, #2712, .F. ) ;
#13457=CARTESIAN_POINT ( 'NONE',  ( 4.182528737366220106, 166.7840834110302808, 323.5943587238651276 ) ) ;
#13469=ADVANCED_FACE ( 'NONE', ( #279, #22632 ), #5206, .F. ) ;
#13482=DIRECTION ( 'NONE',  ( -0.01292394549866731843, -0.005513023399720594006, -0.9999012842304693116 ) ) ;
#13489=VERTEX_POINT ( 'NONE', #10954 ) ;
#13599=CARTESIAN_POINT ( 'NONE',  ( -3.468421381707180728, 158.8820161015420354, 323.7368175311311802 ) ) ;
#13668=DIRECTION ( 'NONE',  ( -0.1136178953597573593, 0.9935164314186355483, -0.004009283626633517415 ) ) ;
#13680=FACE_OUTER_BOUND ( 'NONE', #22074, .T. ) ;
#13702=EDGE_CURVE ( 'NONE', #6945, #10824, #11432, .T. ) ;
#13704=AXIS2_PLACEMENT_3D ( 'NONE', #15472, #6823, #11668 ) ;
#13709=FACE_OUTER_BOUND ( 'NONE', #7486, .T. ) ;
#13715=ORIENTED_EDGE ( 'NONE', *, *, #11840, .T. ) ;
#13717=CARTESIAN_POINT ( 'NONE',  ( -2.503839020269049254, 159.3664414540641587, 324.7217779040802270 ) ) ;
#13726=CIRCLE ( 'NONE', #11146, 11.00000000000000178 ) ;
#13754=VECTOR ( 'NONE', #12961, 1000.000000000000227 ) ;
#13788=CARTESIAN_POINT ( 'NONE',  ( -4.505147608247620283, 176.8666157021447134, 324.6511568656583222 ) ) ;
#13802=DIRECTION ( 'NONE',  ( -0.9934404589540162256, -0.1135548637187056842, 0.01346653032743081423 ) ) ;
#13854=DIRECTION ( 'NONE',  ( -0.01292394549866731669, -0.005513023399720593139, -0.9999012842304692006 ) ) ;
#13862=ADVANCED_FACE ( 'NONE', ( #13157 ), #20120, .T. ) ;
#13896=DIRECTION ( 'NONE',  ( -0.9934404589540162256, -0.1135548637187056842, 0.01346653032743081423 ) ) ;
#13951=DIRECTION ( 'NONE',  ( -0.01292394549866731843, -0.005513023399720594006, -0.9999012842304693116 ) ) ;
#14000=LINE ( 'NONE', #11831, #20184 ) ;
#14016=DIRECTION ( 'NONE',  ( 0.6933298757296778581, 0.07639711794142929613, -0.7165592535100728799 ) ) ;
#14101=ADVANCED_FACE ( 'NONE', ( #6356 ), #5260, .T. ) ;
#14104=PRODUCT_DEFINITION_CONTEXT ( 'detailed design', #4983, 'design' ) ;
#14144=ORIENTED_EDGE ( 'NONE', *, *, #9067, .F. ) ;
#14147=SHAPE_REPRESENTATION_RELATIONSHIP ( 'NONE' , 'NONE' ,  #9590, #3337 ) ;
#14164=ORIENTED_EDGE ( 'NONE', *, *, #20137, .T. ) ;
#14173=ORIENTED_EDGE ( 'NONE', *, *, #8180, .T. ) ;
#14185=AXIS2_PLACEMENT_3D ( 'NONE', #8821, #20887, #13896 ) ;
#14190=CARTESIAN_POINT ( 'NONE',  ( -6.866741853946069618, 164.5525188853477232, 83.72578275117199098 ) ) ;
#14219=LINE ( 'NONE', #1795, #17011 ) ;
#14222=ORIENTED_EDGE ( 'NONE', *, *, #14369, .F. ) ;
#14224=ORIENTED_EDGE ( 'NONE', *, *, #19016, .T. ) ;
#14252=ORIENTED_EDGE ( 'NONE', *, *, #2357, .F. ) ;
#14289=DIRECTION ( 'NONE',  ( 0.01292394549866731843, 0.005513023399720594006, 0.9999012842304693116 ) ) ;
#14298=ORIENTED_EDGE ( 'NONE', *, *, #6738, .T. ) ;
#14327=ORIENTED_EDGE ( 'NONE', *, *, #16442, .T. ) ;
#14343=PRODUCT_DEFINITION_FORMATION_WITH_SPECIFIED_SOURCE ( 'ANY', '', #8650, .NOT_KNOWN. ) ;
#14359=CARTESIAN_POINT ( 'NONE',  ( 14.76142725739638273, 167.8843352801436026, 296.4488922160406332 ) ) ;
#14369=EDGE_CURVE ( 'NONE', #11822, #3438, #7871, .T. ) ;
#14387=MECHANICAL_DESIGN_GEOMETRIC_PRESENTATION_REPRESENTATION('',(#1526),#7140);
#14396=VERTEX_POINT ( 'NONE', #6145 ) ;
#14438=PLANE ( 'NONE',  #16661 ) ;
#14448=FACE_OUTER_BOUND ( 'NONE', #10392, .T. ) ;
#14452=ORIENTED_EDGE ( 'NONE', *, *, #13184, .T. ) ;
#14489=EDGE_CURVE ( 'NONE', #9463, #4261, #3092, .T. ) ;
#14491=AXIS2_PLACEMENT_3D ( 'NONE', #19927, #16852, #8110 ) ;
#14538=FACE_OUTER_BOUND ( 'NONE', #18829, .T. ) ;
#14606=PLANE ( 'NONE',  #12417 ) ;
#14669=AXIS2_PLACEMENT_3D ( 'NONE', #12579, #7272, #17982 ) ;
#14708=EDGE_LOOP ( 'NONE', ( #7979, #2788 ) ) ;
#14733=VECTOR ( 'NONE', #21047, 1000.000000000000114 ) ;
#14776=DIRECTION ( 'NONE',  ( -0.01292394549866731149, -0.005513023399720593139, -0.9999012842304692006 ) ) ;
#14796=EDGE_CURVE ( 'NONE', #19373, #6945, #7152, .T. ) ;
#14811=( LENGTH_UNIT ( ) NAMED_UNIT ( * ) SI_UNIT ( .MILLI., .METRE. ) );
#14824=DIRECTION ( 'NONE',  ( -0.01292394549866731843, -0.005513023399720594006, -0.9999012842304693116 ) ) ;
#14909=DIRECTION ( 'NONE',  ( -0.01292394549866731669, -0.005513023399720593139, -0.9999012842304692006 ) ) ;
#14928=CARTESIAN_POINT ( 'NONE',  ( 7.015576680412771715, 166.1312609306101535, 81.53744875812694204 ) ) ;
#14966=CARTESIAN_POINT ( 'NONE',  ( -6.596016192384672294, 157.5478644388096541, 81.76070674735760235 ) ) ;
#15042=EDGE_LOOP ( 'NONE', ( #4313, #9289 ) ) ;
#15066=ORIENTED_EDGE ( 'NONE', *, *, #22525, .F. ) ;
#15121=DIRECTION ( 'NONE',  ( 0.01292394549866731843, 0.005513023399720594006, 0.9999012842304693116 ) ) ;
#15122=EDGE_LOOP ( 'NONE', ( #17853, #675, #17330, #11397, #12815, #2729, #9742, #2266 ) ) ;
#15182=CARTESIAN_POINT ( 'NONE',  ( 13.10989172854308293, 160.6801362231667269, 299.5102556940336171 ) ) ;
#15187=ORIENTED_EDGE ( 'NONE', *, *, #16379, .T. ) ;
#15303=PLANE ( 'NONE',  #20630 ) ;
#15322=CARTESIAN_POINT ( 'NONE',  ( -1.523404093792848135, 158.5871283748866745, 324.7134023609685869 ) ) ;
#15332=VECTOR ( 'NONE', #260, 1000.000000000000000 ) ;
#15340=B_SPLINE_CURVE_WITH_KNOTS ( 'NONE', 3,
 ( #8308, #22295, #17280, #1544 ),
 .UNSPECIFIED., .F., .F.,
 ( 4, 4 ),
 ( 0.000000000000000000, 0.001461243987308202949 ),
 .UNSPECIFIED. ) ;
#15342=FILL_AREA_STYLE ('',( #4202 ) ) ;
#15365=AXIS2_PLACEMENT_3D ( 'NONE', #7801, #9401, #4332 ) ;
#15434=ORIENTED_EDGE ( 'NONE', *, *, #10615, .F. ) ;
#15472=CARTESIAN_POINT ( 'NONE',  ( 4.195452682864886818, 166.7895964344300239, 324.5942600080955458 ) ) ;
#15516=CARTESIAN_POINT ( 'NONE',  ( 4.195452682864886818, 166.7895964344300239, 324.5942600080955458 ) ) ;
#15523=ORIENTED_EDGE ( 'NONE', *, *, #9670, .F. ) ;
#15528=VERTEX_POINT ( 'NONE', #18001 ) ;
#15628=CARTESIAN_POINT ( 'NONE',  ( -3.394716948004860235, 173.8043418968527192, 324.3209156142289658 ) ) ;
#15638=CARTESIAN_POINT ( 'NONE',  ( -4.705417692162559895, 172.6766985167115820, 324.0106643627350422 ) ) ;
#15689=DIRECTION ( 'NONE',  ( -0.9934404589540162256, -0.1135548637187056842, 0.01346653032743081423 ) ) ;
#15760=LINE ( 'NONE', #4, #17830 ) ;
#15833=EDGE_CURVE ( 'NONE', #22352, #12132, #14000, .T. ) ;
#15836=EDGE_LOOP ( 'NONE', ( #3902, #8414, #22169, #293 ) ) ;
#15876=LINE ( 'NONE', #21127, #6029 ) ;
#15950=AXIS2_PLACEMENT_3D ( 'NONE', #16281, #19253, #3517 ) ;
#15999=LINE ( 'NONE', #21671, #11578 ) ;
#16018=ADVANCED_FACE ( 'NONE', ( #14448 ), #17655, .F. ) ;
#16026=FACE_OUTER_BOUND ( 'NONE', #15042, .T. ) ;
#16033=ORIENTED_EDGE ( 'NONE', *, *, #12181, .T. ) ;
#16045=EDGE_CURVE ( 'NONE', #18202, #16236, #17993, .T. ) ;
#16051=VERTEX_POINT ( 'NONE', #17536 ) ;
#16053=DIRECTION ( 'NONE',  ( -0.9934404589540163366, -0.1135548637187053511, 0.01346653032743023309 ) ) ;
#16099=ORIENTED_EDGE ( 'NONE', *, *, #3005, .T. ) ;
#16125=CARTESIAN_POINT ( 'NONE',  ( -3.593002051346241288, 173.4481159825171233, 324.6582153119202871 ) ) ;
#16165=CIRCLE ( 'NONE', #17241, 10.00000000000005684 ) ;
#16176=LINE ( 'NONE', #17894, #7999 ) ;
#16210=DIRECTION ( 'NONE',  ( 0.9934404589540163366, 0.1135548637187051429, -0.01346653032743023309 ) ) ;
#16212=PLANE ( 'NONE',  #22081 ) ;
#16236=VERTEX_POINT ( 'NONE', #6138 ) ;
#16260=ORIENTED_EDGE ( 'NONE', *, *, #6526, .T. ) ;
#16266=ORIENTED_EDGE ( 'NONE', *, *, #7109, .T. ) ;
#16281=CARTESIAN_POINT ( 'NONE',  ( 11.66102052791742594, 176.1941894196976932, 323.4458143052556238 ) ) ;
#16301=CARTESIAN_POINT ( 'NONE',  ( 11.61857788991896179, 160.0893180226940444, 324.5352569096220918 ) ) ;
#16332=AXIS2_PLACEMENT_3D ( 'NONE', #3143, #1438, #20938 ) ;
#16334=ORIENTED_EDGE ( 'NONE', *, *, #13060, .T. ) ;
#16363=DIRECTION ( 'NONE',  ( -0.01292394549866731843, -0.005513023399720594006, -0.9999012842304693116 ) ) ;
#16379=EDGE_CURVE ( 'NONE', #11822, #15528, #797, .T. ) ;
#16385=CONICAL_SURFACE ( 'NONE', #12701, 11.00000000000000178, 0.7853981633974346233 ) ;
#16425=DIRECTION ( 'NONE',  ( -0.1136178953597577479, 0.9935164314186355483, -0.004009283626633511344 ) ) ;
#16442=EDGE_CURVE ( 'NONE', #1989, #2768, #15340, .T. ) ;
#16488=CARTESIAN_POINT ( 'NONE',  ( 2.945655833907555810, 177.7182771800350167, 324.5501578882025910 ) ) ;
#16568=VERTEX_POINT ( 'NONE', #14190 ) ;
#16630=ORIENTED_EDGE ( 'NONE', *, *, #2356, .F. ) ;
#16657=AXIS2_PLACEMENT_3D ( 'NONE', #1838, #17714, #13802 ) ;
#16661=AXIS2_PLACEMENT_3D ( 'NONE', #17418, #9108, #2012 ) ;
#16669=AXIS2_PLACEMENT_3D ( 'NONE', #17609, #3808, #19200 ) ;
#16703=CARTESIAN_POINT ( 'NONE',  ( -3.227672524189195702, 173.4898748461659750, 324.6532631065690566 ) ) ;
#16736=CARTESIAN_POINT ( 'NONE',  ( 5.047586898063077143, 159.3382231987902173, 324.6243296352952825 ) ) ;
#16761=ORIENTED_EDGE ( 'NONE', *, *, #9993, .T. ) ;
#16766=CARTESIAN_POINT ( 'NONE',  ( 3.833582208902202471, 166.6352317792378415, 296.5970240496424708 ) ) ;
#16811=CARTESIAN_POINT ( 'NONE',  ( -1.788039671088772931, 157.5463400564191545, 323.7224625657159436 ) ) ;
#16827=DIRECTION ( 'NONE',  ( -0.01292394549866731669, -0.005513023399720593139, -0.9999012842304692006 ) ) ;
#16852=DIRECTION ( 'NONE',  ( 0.01292394549866731149, 0.005513023399720593139, 0.9999012842304692006 ) ) ;
#16896=PLANE ( 'NONE',  #11403 ) ;
#16926=CARTESIAN_POINT ( 'NONE',  ( 11.35084583594941066, 176.0618768581043980, 299.4481834837243355 ) ) ;
#16932=CYLINDRICAL_SURFACE ( 'NONE', #1429, 11.00000000000000178 ) ;
#17011=VECTOR ( 'NONE', #5104, 1000.000000000000114 ) ;
#17026=VECTOR ( 'NONE', #21856, 1000.000000000000114 ) ;
#17044=VECTOR ( 'NONE', #12948, 1000.000000000000000 ) ;
#17079=ADVANCED_FACE ( 'NONE', ( #20517 ), #18688, .T. ) ;
#17128=ORIENTED_EDGE ( 'NONE', *, *, #2712, .T. ) ;
#17161=CARTESIAN_POINT ( 'NONE',  ( -5.365183637746670620, 172.6234054757072727, 299.6832001106340613 ) ) ;
#17228=CARTESIAN_POINT ( 'NONE',  ( -4.356009107694418958, 172.5947582827599831, 324.3400096493597289 ) ) ;
#17241=AXIS2_PLACEMENT_3D ( 'NONE', #20915, #4831, #5290 ) ;
#17280=CARTESIAN_POINT ( 'NONE',  ( 12.73831384893346197, 160.9807657804660153, 324.1830962737362256 ) ) ;
#17294=VECTOR ( 'NONE', #16053, 1000.000000000000000 ) ;
#17299=VECTOR ( 'NONE', #16827, 1000.000000000000114 ) ;
#17329=CARTESIAN_POINT ( 'NONE',  ( 13.42006642051110177, 160.8124487847600221, 323.5078865155649055 ) ) ;
#17330=ORIENTED_EDGE ( 'NONE', *, *, #29, .T. ) ;
#17346=VERTEX_POINT ( 'NONE', #7024 ) ;
#17348=CARTESIAN_POINT ( 'NONE',  ( 10.89474438599883221, 174.2127514147958891, 324.4667421121108646 ) ) ;
#17360=DIRECTION ( 'NONE',  ( 0.9934404589540163366, 0.1135548637187057813, -0.01346653032742924430 ) ) ;
#17369=EDGE_CURVE ( 'NONE', #10824, #2768, #16165, .T. ) ;
#17418=CARTESIAN_POINT ( 'NONE',  ( 13.28235005706528682, 159.1720975239875884, 299.5163413053770682 ) ) ;
#17477=CARTESIAN_POINT ( 'NONE',  ( -3.468421381707180728, 158.8820161015420354, 323.7368175311311802 ) ) ;
#17488=ORIENTED_EDGE ( 'NONE', *, *, #3273, .F. ) ;
#17536=CARTESIAN_POINT ( 'NONE',  ( 10.89474438599883221, 174.2127514147958891, 324.4667421121108646 ) ) ;
#17595=DIRECTION ( 'NONE',  ( -0.01292394549866731843, -0.005513023399720594006, -0.9999012842304693116 ) ) ;
#17609=CARTESIAN_POINT ( 'NONE',  ( 1.080781817686064405, 165.4609577950973573, 83.61805050855254251 ) ) ;
#17645=CARTESIAN_POINT ( 'NONE',  ( 4.182528737366220106, 166.7840834110302808, 323.5943587238651276 ) ) ;
#17655=PLANE ( 'NONE',  #7745 ) ;
#17670=COLOUR_RGB ( '', 0.09019608, 0.27058824, 0.51372549) ;
#17673=ORIENTED_EDGE ( 'NONE', *, *, #13060, .F. ) ;
#17707=AXIS2_PLACEMENT_3D ( 'NONE', #18066, #250, #12429 ) ;
#17714=DIRECTION ( 'NONE',  ( -0.01292394549866731843, -0.005513023399720594006, -0.9999012842304693116 ) ) ;
#17742=LINE ( 'NONE', #1987, #15332 ) ;
#17817=PLANE ( 'NONE',  #12960 ) ;
#17830=VECTOR ( 'NONE', #7006, 1000.000000000000114 ) ;
#17853=ORIENTED_EDGE ( 'NONE', *, *, #13702, .T. ) ;
#17855=ORIENTED_EDGE ( 'NONE', *, *, #13702, .F. ) ;
#17894=CARTESIAN_POINT ( 'NONE',  ( -6.847138702882150874, 173.1019677278035829, 81.67819396028960455 ) ) ;
#17974=ORIENTED_EDGE ( 'NONE', *, *, #13250, .T. ) ;
#17981=CARTESIAN_POINT ( 'NONE',  ( 5.047586898063077143, 159.3382231987902173, 324.6243296352952825 ) ) ;
#17982=DIRECTION ( 'NONE',  ( -0.9934404589540162256, -0.1135548637187056842, 0.01346653032743081423 ) ) ;
#17993=LINE ( 'NONE', #1903, #17294 ) ;
#18001=CARTESIAN_POINT ( 'NONE',  ( 11.52330416447161276, 174.5538381589252594, 299.4542690950677297 ) ) ;
#18034=DIRECTION ( 'NONE',  ( 0.01292394549866731149, 0.005513023399720593139, 0.9999012842304692006 ) ) ;
#18035=DIRECTION ( 'NONE',  ( 0.7116070947332637786, 0.08419371040299428177, 0.6975147036829121294 ) ) ;
#18066=CARTESIAN_POINT ( 'NONE',  ( 1.054933926688728762, 165.4499317482979279, 81.61824794009152129 ) ) ;
#18097=CARTESIAN_POINT ( 'NONE',  ( 3.833582208902202471, 166.6352317792378415, 296.5970240496424708 ) ) ;
#18113=CARTESIAN_POINT ( 'NONE',  ( 3.833582208902202471, 166.6352317792378415, 296.5970240496424708 ) ) ;
#18147=AXIS2_PLACEMENT_3D ( 'NONE', #5503, #17595, #5382 ) ;
#18202=VERTEX_POINT ( 'NONE', #343 ) ;
#18208=FACE_OUTER_BOUND ( 'NONE', #15122, .T. ) ;
#18443=PRODUCT_DEFINITION ( 'UNKNOWN', '', #14343, #14104 ) ;
#18504=CARTESIAN_POINT ( 'NONE',  ( 10.85296234298433404, 174.5781088801995793, 324.4652677311569278 ) ) ;
#18553=CARTESIAN_POINT ( 'NONE',  ( -5.055008945778654450, 172.7557180373005679, 323.6808309321652928 ) ) ;
#18567=LINE ( 'NONE', #6277, #13754 ) ;
#18599=EDGE_LOOP ( 'NONE', ( #1187, #13225, #16099, #8597 ) ) ;
#18611=CARTESIAN_POINT ( 'NONE',  ( 1.054933926688728762, 165.4499317482979279, 81.61824794009152129 ) ) ;
#18657=EDGE_LOOP ( 'NONE', ( #19562, #10192, #14144, #7608, #8638, #16334, #17128, #19652, #3803, #3330, #22258, #595 ) ) ;
#18688=PLANE ( 'NONE',  #7413 ) ;
#18760=SURFACE_STYLE_USAGE ( .BOTH. , #7773 ) ;
#18804=VECTOR ( 'NONE', #10666, 1000.000000000000000 ) ;
#18813=DIRECTION ( 'NONE',  ( 0.01292394549866731149, 0.005513023399720593139, 0.9999012842304692006 ) ) ;
#18829=EDGE_LOOP ( 'NONE', ( #2815, #12659, #6349, #17855 ) ) ;
#18881=ORIENTED_EDGE ( 'NONE', *, *, #93, .F. ) ;
#18914=EDGE_LOOP ( 'NONE', ( #20301, #2268, #20386, #19242 ) ) ;
#18927=CARTESIAN_POINT ( 'NONE',  ( -3.295963053184979508, 157.3739774023628968, 323.7429031424746881 ) ) ;
#18949=DIRECTION ( 'NONE',  ( -0.1136178953597573593, 0.9935164314186355483, -0.004009283626633517415 ) ) ;
#18988=CIRCLE ( 'NONE', #3236, 8.000000000000003553 ) ;
#18997=DIRECTION ( 'NONE',  ( -0.9934404589540162256, -0.1135548637187056842, 0.01346653032743081423 ) ) ;
#19003=LINE ( 'NONE', #6833, #12512 ) ;
#19010=CIRCLE ( 'NONE', #20845, 5.999999999999952038 ) ;
#19016=EDGE_CURVE ( 'NONE', #10791, #16568, #9158, .T. ) ;
#19038=ADVANCED_FACE ( 'NONE', ( #11130 ), #17817, .T. ) ;
#19045=CARTESIAN_POINT ( 'NONE',  ( 11.20671232108558257, 174.3736497049977174, 324.1290499907220237 ) ) ;
#19047=DIRECTION ( 'NONE',  ( 0.1136178953597573732, -0.9935164314186356593, 0.004009283626633518283 ) ) ;
#19071=AXIS2_PLACEMENT_3D ( 'NONE', #17645, #21182, #10860 ) ;
#19110=AXIS2_PLACEMENT_3D ( 'NONE', #18611, #20335, #2875 ) ;
#19131=ORIENTED_EDGE ( 'NONE', *, *, #5330, .F. ) ;
#19136=CARTESIAN_POINT ( 'NONE',  ( -4.029718584172675477, 174.3038068289426690, 299.6566739225319225 ) ) ;
#19177=EDGE_CURVE ( 'NONE', #10848, #5715, #104, .T. ) ;
#19200=DIRECTION ( 'NONE',  ( 0.9934404589540162256, 0.1135548637187059617, -0.01346653032742970747 ) ) ;
#19242=ORIENTED_EDGE ( 'NONE', *, *, #16045, .F. ) ;
#19253=DIRECTION ( 'NONE',  ( -0.07120137477123651693, 0.7064205021071690016, 0.7042019869563996837 ) ) ;
#19364=CARTESIAN_POINT ( 'NONE',  ( 10.29247160983360843, 159.4782971220276693, 81.53177573179129922 ) ) ;
#19373=VERTEX_POINT ( 'NONE', #12266 ) ;
#19401=DIRECTION ( 'NONE',  ( -0.1136178953597573593, 0.9935164314186355483, -0.004009283626633517415 ) ) ;
#19440=CIRCLE ( 'NONE', #2931, 11.00000000000000178 ) ;
#19448=FACE_OUTER_BOUND ( 'NONE', #224, .T. ) ;
#19450=CARTESIAN_POINT ( 'NONE',  ( 3.833582208902202471, 166.6352317792378415, 296.5970240496424708 ) ) ;
#19505=CARTESIAN_POINT ( 'NONE',  ( -3.719543892204659752, 174.4361193905359642, 323.6543047440632108 ) ) ;
#19507=EDGE_LOOP ( 'NONE', ( #10866, #17488, #865, #2082 ) ) ;
#19562=ORIENTED_EDGE ( 'NONE', *, *, #16379, .F. ) ;
#19572=AXIS2_PLACEMENT_3D ( 'NONE', #4049, #19665, #21727 ) ;
#19625=FACE_OUTER_BOUND ( 'NONE', #6221, .T. ) ;
#19652=ORIENTED_EDGE ( 'NONE', *, *, #1841, .F. ) ;
#19654=CARTESIAN_POINT ( 'NONE',  ( 4.195452682864886818, 166.7895964344300239, 324.5942600080955458 ) ) ;
#19665=DIRECTION ( 'NONE',  ( 0.01292394549866731149, 0.005513023399720593139, 0.9999012842304692006 ) ) ;
#19720=ORIENTED_EDGE ( 'NONE', *, *, #9670, .T. ) ;
#19726=ORIENTED_EDGE ( 'NONE', *, *, #5846, .F. ) ;
#19731=EDGE_CURVE ( 'NONE', #16051, #11842, #1959, .T. ) ;
#19749=FACE_OUTER_BOUND ( 'NONE', #18657, .T. ) ;
#19910=ORIENTED_EDGE ( 'NONE', *, *, #14796, .F. ) ;
#19927=CARTESIAN_POINT ( 'NONE',  ( 3.872354045398203937, 166.6517708494369856, 299.5967279023338392 ) ) ;
#19943=CARTESIAN_POINT ( 'NONE',  ( 11.35084583594941066, 176.0618768581043980, 299.4481834837243355 ) ) ;
#19991=ADVANCED_FACE ( 'NONE', ( #18208 ), #2455, .F. ) ;
#20025=DIRECTION ( 'NONE',  ( -0.9934404589540162256, -0.1135548637187056842, 0.01346653032743081423 ) ) ;
#20038=DIRECTION ( 'NONE',  ( 0.01292394549866731669, 0.005513023399720593139, 0.9999012842304692006 ) ) ;
#20085=DIRECTION ( 'NONE',  ( -0.1136178953597573593, 0.9935164314186355483, -0.004009283626633517415 ) ) ;
#20088=DIRECTION ( 'NONE',  ( -0.9934404589540162256, -0.1135548637187056842, 0.01346653032743081423 ) ) ;
#20120=PLANE ( 'NONE',  #15950 ) ;
#20137=EDGE_CURVE ( 'NONE', #16568, #12132, #1609, .T. ) ;
#20182=AXIS2_PLACEMENT_3D ( 'NONE', #5646, #12340, #7153 ) ;
#20184=VECTOR ( 'NONE', #12161, 1000.000000000000114 ) ;
#20191=ORIENTED_EDGE ( 'NONE', *, *, #10949, .F. ) ;
#20301=ORIENTED_EDGE ( 'NONE', *, *, #6526, .F. ) ;
#20335=DIRECTION ( 'NONE',  ( -0.01292394549866731843, -0.005513023399720594006, -0.9999012842304693116 ) ) ;
#20342=LINE ( 'NONE', #20553, #8514 ) ;
#20352=ORIENTED_EDGE ( 'NONE', *, *, #8776, .T. ) ;
#20386=ORIENTED_EDGE ( 'NONE', *, *, #3297, .F. ) ;
#20430=CARTESIAN_POINT ( 'NONE',  ( 11.83347885643962982, 174.6861507205185546, 323.4518999165990181 ) ) ;
#20490=CARTESIAN_POINT ( 'NONE',  ( 11.78110588053433716, 167.5436706889874756, 296.4892918070229939 ) ) ;
#20508=VECTOR ( 'NONE', #7359, 1000.000000000000114 ) ;
#20517=FACE_OUTER_BOUND ( 'NONE', #14708, .T. ) ;
#20553=CARTESIAN_POINT ( 'NONE',  ( -3.606137745152995233, 157.2416648407696016, 299.7452723209433998 ) ) ;
#20594=AXIS2_PLACEMENT_3D ( 'NONE', #18097, #7385, #8995 ) ;
#20614=CARTESIAN_POINT ( 'NONE',  ( 9.914309459522627321, 174.9920644939733734, 324.4751176552225616 ) ) ;
#20630=AXIS2_PLACEMENT_3D ( 'NONE', #13788, #14016, #19047 ) ;
#20658=EDGE_CURVE ( 'NONE', #1989, #2734, #5693, .T. ) ;
#20688=VERTEX_POINT ( 'NONE', #9136 ) ;
#20768=ADVANCED_FACE ( 'NONE', ( #4302 ), #771, .T. ) ;
#20790=EDGE_CURVE ( 'NONE', #12915, #19373, #18567, .T. ) ;
#20829=CARTESIAN_POINT ( 'NONE',  ( 9.842922453853201858, 175.8895142040481403, 299.4686240604829663 ) ) ;
#20845=AXIS2_PLACEMENT_3D ( 'NONE', #11525, #9795, #10134 ) ;
#20850=EDGE_CURVE ( 'NONE', #20688, #11842, #13015, .T. ) ;
#20855=VERTEX_POINT ( 'NONE', #4870 ) ;
#20877=VECTOR ( 'NONE', #13668, 1000.000000000000227 ) ;
#20887=DIRECTION ( 'NONE',  ( -0.01292394549866731843, -0.005513023399720594006, -0.9999012842304693116 ) ) ;
#20915=CARTESIAN_POINT ( 'NONE',  ( 4.195452682864886818, 166.7895964344300239, 324.5942600080955458 ) ) ;
#20938=DIRECTION ( 'NONE',  ( 0.9934404589540162256, 0.1135548637187056842, -0.01346653032743081423 ) ) ;
#20956=CARTESIAN_POINT ( 'NONE',  ( -3.606137745152995233, 157.2416648407696016, 299.7452723209433998 ) ) ;
#20981=ORIENTED_EDGE ( 'NONE', *, *, #7109, .F. ) ;
#21001=CIRCLE ( 'NONE', #11122, 8.000000000000003553 ) ;
#21023=EDGE_CURVE ( 'NONE', #20688, #10848, #747, .T. ) ;
#21047=DIRECTION ( 'NONE',  ( -0.01292394549866731669, -0.005513023399720593139, -0.9999012842304692006 ) ) ;
#21127=CARTESIAN_POINT ( 'NONE',  ( 13.28235005706528682, 159.1720975239875884, 299.5163413053770682 ) ) ;
#21182=DIRECTION ( 'NONE',  ( -0.01292394549866731843, -0.005513023399720594006, -0.9999012842304693116 ) ) ;
#21310=ORIENTED_EDGE ( 'NONE', *, *, #693, .F. ) ;
#21350=DIRECTION ( 'NONE',  ( -0.01292394549866731669, -0.005513023399720593139, -0.9999012842304692006 ) ) ;
#21470=CARTESIAN_POINT ( 'NONE',  ( -3.558528459570483360, 174.1198169369959317, 323.9878838343831262 ) ) ;
#21518=CARTESIAN_POINT ( 'NONE',  ( -3.227672524189195702, 173.4898748461659750, 324.6532631065690566 ) ) ;
#21558=DIRECTION ( 'NONE',  ( 0.01292394549866731149, 0.005513023399720593139, 0.9999012842304692006 ) ) ;
#21560=CIRCLE ( 'NONE', #15365, 5.999999999999952038 ) ;
#21594=EDGE_LOOP ( 'NONE', ( #15434, #7798, #9072, #13385 ) ) ;
#21671=CARTESIAN_POINT ( 'NONE',  ( -6.892589744943404817, 164.5414928385482654, 81.72598018271095555 ) ) ;
#21727=DIRECTION ( 'NONE',  ( 0.9934404589540163366, 0.1135548637187051429, -0.01346653032743023309 ) ) ;
#21728=DIRECTION ( 'NONE',  ( -0.9934404589540163366, -0.1135548637187051429, 0.01346653032743023309 ) ) ;
#21774=DIRECTION ( 'NONE',  ( 0.01292394549866731843, 0.005513023399720594006, 0.9999012842304693116 ) ) ;
#21856=DIRECTION ( 'NONE',  ( 0.9934404589540162256, 0.1135548637187055315, -0.01346653032743023309 ) ) ;
#21930=ORIENTED_EDGE ( 'NONE', *, *, #21023, .T. ) ;
#21934=ORIENTED_EDGE ( 'NONE', *, *, #13338, .T. ) ;
#21953=CLOSED_SHELL ( 'NONE', ( #1565, #22599, #5285, #4339, #19991, #1791, #4300, #13469, #7576, #3457, #6538, #16018, #20768, #10973, #17079, #19038, #21970, #10612, #13862, #7924, #14101, #4490, #8122, #7122, #10465 ) ) ;
#21970=ADVANCED_FACE ( 'NONE', ( #13680 ), #16896, .T. ) ;
#22034=VECTOR ( 'NONE', #6969, 1000.000000000000114 ) ;
#22072=DIRECTION ( 'NONE',  ( -0.01292394549866731843, -0.005513023399720594006, -0.9999012842304693116 ) ) ;
#22073=DIRECTION ( 'NONE',  ( 0.9934404589540162256, 0.1135548637187056842, -0.01346653032743081423 ) ) ;
#22074=EDGE_LOOP ( 'NONE', ( #16761, #16033, #3183, #13715 ) ) ;
#22081=AXIS2_PLACEMENT_3D ( 'NONE', #11006, #18035, #2283 ) ;
#22104=CIRCLE ( 'NONE', #7839, 11.00000000000000178 ) ;
#22132=EDGE_CURVE ( 'NONE', #14396, #1325, #9658, .T. ) ;
#22157=LINE ( 'NONE', #14966, #2244 ) ;
#22169=ORIENTED_EDGE ( 'NONE', *, *, #16442, .F. ) ;
#22258=ORIENTED_EDGE ( 'NONE', *, *, #10949, .T. ) ;
#22295=CARTESIAN_POINT ( 'NONE',  ( 13.07910534688314819, 160.8951497186004076, 323.8457538311976123 ) ) ;
#22337=LINE ( 'NONE', #17329, #6411 ) ;
#22352=VERTEX_POINT ( 'NONE', #20490 ) ;
#22441=ORIENTED_EDGE ( 'NONE', *, *, #22132, .T. ) ;
#22476=CARTESIAN_POINT ( 'NONE',  ( -4.006862498311197562, 172.5094284590153393, 324.6687400670222701 ) ) ;
#22500=DIRECTION ( 'NONE',  ( -0.9934404589540162256, -0.1135548637187059617, 0.01346653032742970747 ) ) ;
#22519=AXIS2_PLACEMENT_3D ( 'NONE', #2442, #4146, #2328 ) ;
#22525=EDGE_CURVE ( 'NONE', #11778, #17346, #22157, .T. ) ;
#22565=APPLICATION_CONTEXT ( 'automotive_design' ) ;
#22599=ADVANCED_FACE ( 'NONE', ( #9784 ), #13359, .T. ) ;
#22623=ORIENTED_EDGE ( 'NONE', *, *, #12885, .F. ) ;
#22632=FACE_OUTER_BOUND ( 'NONE', #2267, .T. ) ;
#22637=CARTESIAN_POINT ( 'NONE',  ( 10.15309714582121714, 176.0218267656414355, 323.4662548820142547 ) ) ;
ENDSEC;
END-ISO-10303-21;
